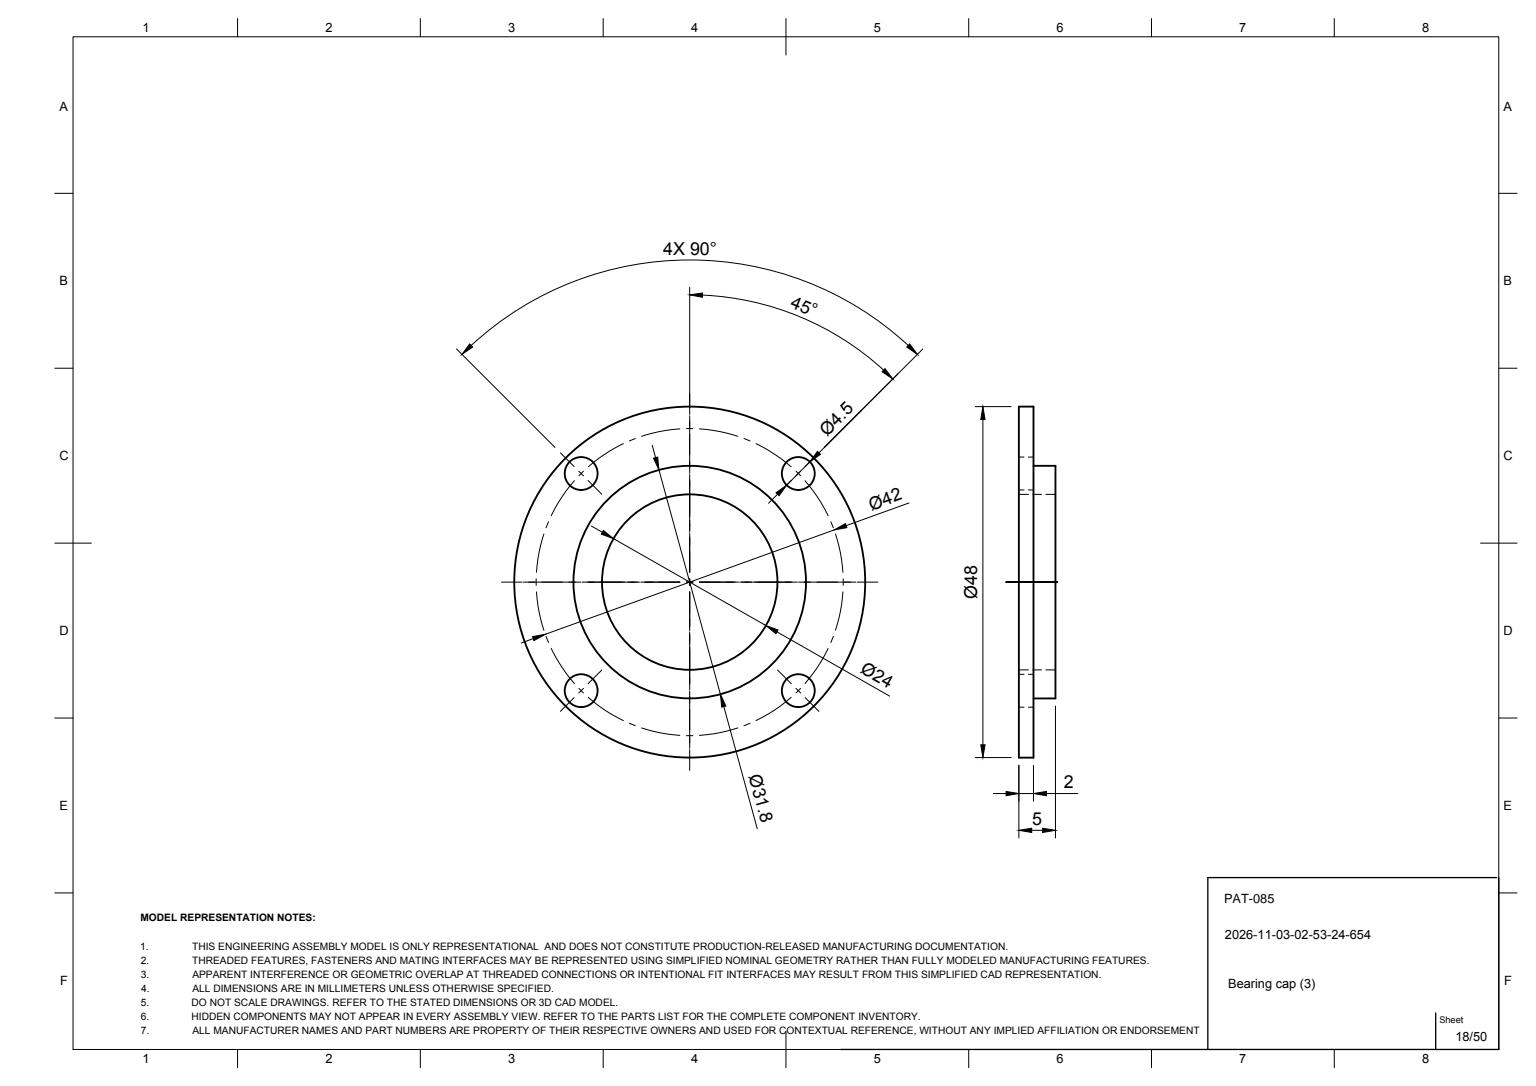
ISO-10303-21;
HEADER;
/* Generated by software containing ST-Developer
 * from STEP Tools, Inc. (www.steptools.com) 
 */

FILE_DESCRIPTION(
/* description */ ('Rack and pinion manual slide'),
/* implementation_level */ '2;1');

FILE_NAME(
/* name */ 'Bearing cap (3).step',
/* time_stamp */ '2026-10-28T03:22:49-07:00',
/* author */ (''),
/* organization */ (''),
/* preprocessor_version */ 'ST-DEVELOPER v20.2',
/* originating_system */ 'Autodesk Translation Framework v15.17.0.0',
/* authorisation */ '');

FILE_SCHEMA (('AUTOMOTIVE_DESIGN { 1 0 10303 214 3 1 1 }'));
ENDSEC;

DATA;
#10=MECHANICAL_DESIGN_GEOMETRIC_PRESENTATION_REPRESENTATION('',(#745),#34851);
#653=SHAPE_REPRESENTATION_RELATIONSHIP('SRR','None',#35088,#699);
#699=ADVANCED_BREP_SHAPE_REPRESENTATION('',(#798),#34813);
#745=STYLED_ITEM('',(#35411),#798);
#798=MANIFOLD_SOLID_BREP('Body1',#13765);
#946=FACE_BOUND('',#2537,.T.);
#947=FACE_BOUND('',#2541,.T.);
#948=FACE_BOUND('',#2542,.T.);
#949=FACE_BOUND('',#2543,.T.);
#950=FACE_BOUND('',#2544,.T.);
#951=FACE_BOUND('',#2545,.T.);
#952=FACE_BOUND('',#2547,.T.);
#953=FACE_BOUND('',#2548,.T.);
#954=FACE_BOUND('',#2549,.T.);
#955=FACE_BOUND('',#2550,.T.);
#956=FACE_BOUND('',#2551,.T.);
#1125=PLANE('',#14618);
#1126=PLANE('',#14625);
#1127=PLANE('',#14626);
#1679=FACE_OUTER_BOUND('',#2531,.T.);
#1680=FACE_OUTER_BOUND('',#2532,.T.);
#1681=FACE_OUTER_BOUND('',#2533,.T.);
#1682=FACE_OUTER_BOUND('',#2534,.T.);
#1683=FACE_OUTER_BOUND('',#2535,.T.);
#1684=FACE_OUTER_BOUND('',#2536,.T.);
#1685=FACE_OUTER_BOUND('',#2538,.T.);
#1686=FACE_OUTER_BOUND('',#2539,.T.);
#1687=FACE_OUTER_BOUND('',#2540,.T.);
#1688=FACE_OUTER_BOUND('',#2546,.T.);
#2531=EDGE_LOOP('',(#9900,#9901,#9902,#9903));
#2532=EDGE_LOOP('',(#9904,#9905,#9906,#9907));
#2533=EDGE_LOOP('',(#9908,#9909,#9910,#9911));
#2534=EDGE_LOOP('',(#9912,#9913,#9914,#9915));
#2535=EDGE_LOOP('',(#9916,#9917,#9918,#9919));
#2536=EDGE_LOOP('',(#9920));
#2537=EDGE_LOOP('',(#9921));
#2538=EDGE_LOOP('',(#9922,#9923,#9924,#9925));
#2539=EDGE_LOOP('',(#9926,#9927,#9928,#9929));
#2540=EDGE_LOOP('',(#9930));
#2541=EDGE_LOOP('',(#9931));
#2542=EDGE_LOOP('',(#9932));
#2543=EDGE_LOOP('',(#9933));
#2544=EDGE_LOOP('',(#9934));
#2545=EDGE_LOOP('',(#9935));
#2546=EDGE_LOOP('',(#9936));
#2547=EDGE_LOOP('',(#9937));
#2548=EDGE_LOOP('',(#9938));
#2549=EDGE_LOOP('',(#9939));
#2550=EDGE_LOOP('',(#9940));
#2551=EDGE_LOOP('',(#9941));
#3431=LINE('',#20176,#4722);
#3432=LINE('',#20182,#4723);
#3433=LINE('',#20188,#4724);
#3434=LINE('',#20194,#4725);
#3435=LINE('',#20200,#4726);
#3436=LINE('',#20208,#4727);
#3437=LINE('',#20213,#4728);
#4722=VECTOR('',#16383,0.225);
#4723=VECTOR('',#16390,0.225);
#4724=VECTOR('',#16397,0.225);
#4725=VECTOR('',#16404,0.225);
#4726=VECTOR('',#16411,1.59);
#4727=VECTOR('',#16422,1.2);
#4728=VECTOR('',#16427,2.4);
#5932=CIRCLE('',#14604,0.225);
#5933=CIRCLE('',#14605,0.225);
#5934=CIRCLE('',#14607,0.225);
#5935=CIRCLE('',#14608,0.225);
#5936=CIRCLE('',#14610,0.225);
#5937=CIRCLE('',#14611,0.225);
#5938=CIRCLE('',#14613,0.225);
#5939=CIRCLE('',#14614,0.225);
#5940=CIRCLE('',#14616,1.59);
#5941=CIRCLE('',#14617,1.59);
#5942=CIRCLE('',#14619,1.2);
#5943=CIRCLE('',#14621,1.2);
#5944=CIRCLE('',#14623,2.4);
#5945=CIRCLE('',#14624,2.4);
#6446=VERTEX_POINT('',#20173);
#6447=VERTEX_POINT('',#20175);
#6448=VERTEX_POINT('',#20179);
#6449=VERTEX_POINT('',#20181);
#6450=VERTEX_POINT('',#20185);
#6451=VERTEX_POINT('',#20187);
#6452=VERTEX_POINT('',#20191);
#6453=VERTEX_POINT('',#20193);
#6454=VERTEX_POINT('',#20197);
#6455=VERTEX_POINT('',#20199);
#6456=VERTEX_POINT('',#20203);
#6457=VERTEX_POINT('',#20206);
#6458=VERTEX_POINT('',#20210);
#6459=VERTEX_POINT('',#20212);
#7762=EDGE_CURVE('',#6446,#6446,#5932,.T.);
#7763=EDGE_CURVE('',#6446,#6447,#3431,.T.);
#7764=EDGE_CURVE('',#6447,#6447,#5933,.T.);
#7765=EDGE_CURVE('',#6448,#6448,#5934,.T.);
#7766=EDGE_CURVE('',#6448,#6449,#3432,.T.);
#7767=EDGE_CURVE('',#6449,#6449,#5935,.T.);
#7768=EDGE_CURVE('',#6450,#6450,#5936,.T.);
#7769=EDGE_CURVE('',#6450,#6451,#3433,.T.);
#7770=EDGE_CURVE('',#6451,#6451,#5937,.T.);
#7771=EDGE_CURVE('',#6452,#6452,#5938,.T.);
#7772=EDGE_CURVE('',#6452,#6453,#3434,.T.);
#7773=EDGE_CURVE('',#6453,#6453,#5939,.T.);
#7774=EDGE_CURVE('',#6454,#6454,#5940,.T.);
#7775=EDGE_CURVE('',#6454,#6455,#3435,.T.);
#7776=EDGE_CURVE('',#6455,#6455,#5941,.T.);
#7777=EDGE_CURVE('',#6456,#6456,#5942,.T.);
#7778=EDGE_CURVE('',#6457,#6457,#5943,.T.);
#7779=EDGE_CURVE('',#6457,#6456,#3436,.T.);
#7780=EDGE_CURVE('',#6458,#6458,#5944,.T.);
#7781=EDGE_CURVE('',#6458,#6459,#3437,.T.);
#7782=EDGE_CURVE('',#6459,#6459,#5945,.T.);
#9900=ORIENTED_EDGE('',*,*,#7762,.F.);
#9901=ORIENTED_EDGE('',*,*,#7763,.T.);
#9902=ORIENTED_EDGE('',*,*,#7764,.F.);
#9903=ORIENTED_EDGE('',*,*,#7763,.F.);
#9904=ORIENTED_EDGE('',*,*,#7765,.F.);
#9905=ORIENTED_EDGE('',*,*,#7766,.T.);
#9906=ORIENTED_EDGE('',*,*,#7767,.F.);
#9907=ORIENTED_EDGE('',*,*,#7766,.F.);
#9908=ORIENTED_EDGE('',*,*,#7768,.F.);
#9909=ORIENTED_EDGE('',*,*,#7769,.T.);
#9910=ORIENTED_EDGE('',*,*,#7770,.F.);
#9911=ORIENTED_EDGE('',*,*,#7769,.F.);
#9912=ORIENTED_EDGE('',*,*,#7771,.F.);
#9913=ORIENTED_EDGE('',*,*,#7772,.T.);
#9914=ORIENTED_EDGE('',*,*,#7773,.F.);
#9915=ORIENTED_EDGE('',*,*,#7772,.F.);
#9916=ORIENTED_EDGE('',*,*,#7774,.F.);
#9917=ORIENTED_EDGE('',*,*,#7775,.T.);
#9918=ORIENTED_EDGE('',*,*,#7776,.T.);
#9919=ORIENTED_EDGE('',*,*,#7775,.F.);
#9920=ORIENTED_EDGE('',*,*,#7776,.F.);
#9921=ORIENTED_EDGE('',*,*,#7777,.F.);
#9922=ORIENTED_EDGE('',*,*,#7778,.F.);
#9923=ORIENTED_EDGE('',*,*,#7779,.T.);
#9924=ORIENTED_EDGE('',*,*,#7777,.T.);
#9925=ORIENTED_EDGE('',*,*,#7779,.F.);
#9926=ORIENTED_EDGE('',*,*,#7780,.F.);
#9927=ORIENTED_EDGE('',*,*,#7781,.T.);
#9928=ORIENTED_EDGE('',*,*,#7782,.T.);
#9929=ORIENTED_EDGE('',*,*,#7781,.F.);
#9930=ORIENTED_EDGE('',*,*,#7780,.T.);
#9931=ORIENTED_EDGE('',*,*,#7778,.T.);
#9932=ORIENTED_EDGE('',*,*,#7773,.T.);
#9933=ORIENTED_EDGE('',*,*,#7770,.T.);
#9934=ORIENTED_EDGE('',*,*,#7767,.T.);
#9935=ORIENTED_EDGE('',*,*,#7764,.T.);
#9936=ORIENTED_EDGE('',*,*,#7782,.F.);
#9937=ORIENTED_EDGE('',*,*,#7774,.T.);
#9938=ORIENTED_EDGE('',*,*,#7771,.T.);
#9939=ORIENTED_EDGE('',*,*,#7768,.T.);
#9940=ORIENTED_EDGE('',*,*,#7765,.T.);
#9941=ORIENTED_EDGE('',*,*,#7762,.T.);
#12907=CYLINDRICAL_SURFACE('',#14603,0.225);
#12908=CYLINDRICAL_SURFACE('',#14606,0.225);
#12909=CYLINDRICAL_SURFACE('',#14609,0.225);
#12910=CYLINDRICAL_SURFACE('',#14612,0.225);
#12911=CYLINDRICAL_SURFACE('',#14615,1.59);
#12912=CYLINDRICAL_SURFACE('',#14620,1.2);
#12913=CYLINDRICAL_SURFACE('',#14622,2.4);
#13157=ADVANCED_FACE('',(#1679),#12907,.F.);
#13158=ADVANCED_FACE('',(#1680),#12908,.F.);
#13159=ADVANCED_FACE('',(#1681),#12909,.F.);
#13160=ADVANCED_FACE('',(#1682),#12910,.F.);
#13161=ADVANCED_FACE('',(#1683),#12911,.T.);
#13162=ADVANCED_FACE('',(#1684,#946),#1125,.F.);
#13163=ADVANCED_FACE('',(#1685),#12912,.F.);
#13164=ADVANCED_FACE('',(#1686),#12913,.T.);
#13165=ADVANCED_FACE('',(#1687,#947,#948,#949,#950,#951),#1126,.T.);
#13166=ADVANCED_FACE('',(#1688,#952,#953,#954,#955,#956),#1127,.F.);
#13765=CLOSED_SHELL('',(#13157,#13158,#13159,#13160,#13161,#13162,#13163,
#13164,#13165,#13166));
#14602=AXIS2_PLACEMENT_3D('',#20171,#16377,#16378);
#14603=AXIS2_PLACEMENT_3D('',#20172,#16379,#16380);
#14604=AXIS2_PLACEMENT_3D('',#20174,#16381,#16382);
#14605=AXIS2_PLACEMENT_3D('',#20177,#16384,#16385);
#14606=AXIS2_PLACEMENT_3D('',#20178,#16386,#16387);
#14607=AXIS2_PLACEMENT_3D('',#20180,#16388,#16389);
#14608=AXIS2_PLACEMENT_3D('',#20183,#16391,#16392);
#14609=AXIS2_PLACEMENT_3D('',#20184,#16393,#16394);
#14610=AXIS2_PLACEMENT_3D('',#20186,#16395,#16396);
#14611=AXIS2_PLACEMENT_3D('',#20189,#16398,#16399);
#14612=AXIS2_PLACEMENT_3D('',#20190,#16400,#16401);
#14613=AXIS2_PLACEMENT_3D('',#20192,#16402,#16403);
#14614=AXIS2_PLACEMENT_3D('',#20195,#16405,#16406);
#14615=AXIS2_PLACEMENT_3D('',#20196,#16407,#16408);
#14616=AXIS2_PLACEMENT_3D('',#20198,#16409,#16410);
#14617=AXIS2_PLACEMENT_3D('',#20201,#16412,#16413);
#14618=AXIS2_PLACEMENT_3D('',#20202,#16414,#16415);
#14619=AXIS2_PLACEMENT_3D('',#20204,#16416,#16417);
#14620=AXIS2_PLACEMENT_3D('',#20205,#16418,#16419);
#14621=AXIS2_PLACEMENT_3D('',#20207,#16420,#16421);
#14622=AXIS2_PLACEMENT_3D('',#20209,#16423,#16424);
#14623=AXIS2_PLACEMENT_3D('',#20211,#16425,#16426);
#14624=AXIS2_PLACEMENT_3D('',#20214,#16428,#16429);
#14625=AXIS2_PLACEMENT_3D('',#20215,#16430,#16431);
#14626=AXIS2_PLACEMENT_3D('',#20216,#16432,#16433);
#16377=DIRECTION('axis',(0.,0.,1.));
#16378=DIRECTION('refdir',(1.,0.,0.));
#16379=DIRECTION('center_axis',(0.,1.,0.));
#16380=DIRECTION('ref_axis',(1.,0.,0.));
#16381=DIRECTION('center_axis',(0.,1.,0.));
#16382=DIRECTION('ref_axis',(1.,0.,0.));
#16383=DIRECTION('',(0.,1.,0.));
#16384=DIRECTION('center_axis',(0.,-1.,0.));
#16385=DIRECTION('ref_axis',(1.,0.,0.));
#16386=DIRECTION('center_axis',(0.,1.,0.));
#16387=DIRECTION('ref_axis',(1.,0.,0.));
#16388=DIRECTION('center_axis',(0.,1.,0.));
#16389=DIRECTION('ref_axis',(1.,0.,0.));
#16390=DIRECTION('',(0.,1.,0.));
#16391=DIRECTION('center_axis',(0.,-1.,0.));
#16392=DIRECTION('ref_axis',(1.,0.,0.));
#16393=DIRECTION('center_axis',(0.,1.,0.));
#16394=DIRECTION('ref_axis',(1.,0.,0.));
#16395=DIRECTION('center_axis',(0.,1.,0.));
#16396=DIRECTION('ref_axis',(1.,0.,0.));
#16397=DIRECTION('',(0.,1.,0.));
#16398=DIRECTION('center_axis',(0.,-1.,0.));
#16399=DIRECTION('ref_axis',(1.,0.,0.));
#16400=DIRECTION('center_axis',(0.,1.,0.));
#16401=DIRECTION('ref_axis',(1.,0.,0.));
#16402=DIRECTION('center_axis',(0.,1.,0.));
#16403=DIRECTION('ref_axis',(1.,0.,0.));
#16404=DIRECTION('',(0.,1.,0.));
#16405=DIRECTION('center_axis',(0.,-1.,0.));
#16406=DIRECTION('ref_axis',(1.,0.,0.));
#16407=DIRECTION('center_axis',(0.,1.,0.));
#16408=DIRECTION('ref_axis',(1.,0.,0.));
#16409=DIRECTION('center_axis',(0.,1.,0.));
#16410=DIRECTION('ref_axis',(1.,0.,0.));
#16411=DIRECTION('',(0.,-1.,0.));
#16412=DIRECTION('center_axis',(0.,1.,0.));
#16413=DIRECTION('ref_axis',(1.,0.,0.));
#16414=DIRECTION('center_axis',(0.,1.,0.));
#16415=DIRECTION('ref_axis',(1.,0.,0.));
#16416=DIRECTION('center_axis',(0.,-1.,0.));
#16417=DIRECTION('ref_axis',(1.,0.,0.));
#16418=DIRECTION('center_axis',(0.,1.,0.));
#16419=DIRECTION('ref_axis',(1.,0.,0.));
#16420=DIRECTION('center_axis',(0.,-1.,0.));
#16421=DIRECTION('ref_axis',(1.,0.,0.));
#16422=DIRECTION('',(0.,-1.,0.));
#16423=DIRECTION('center_axis',(0.,1.,0.));
#16424=DIRECTION('ref_axis',(1.,0.,0.));
#16425=DIRECTION('center_axis',(0.,1.,0.));
#16426=DIRECTION('ref_axis',(1.,0.,0.));
#16427=DIRECTION('',(0.,-1.,0.));
#16428=DIRECTION('center_axis',(0.,1.,0.));
#16429=DIRECTION('ref_axis',(1.,0.,0.));
#16430=DIRECTION('center_axis',(0.,1.,0.));
#16431=DIRECTION('ref_axis',(1.,0.,0.));
#16432=DIRECTION('center_axis',(0.,1.,0.));
#16433=DIRECTION('ref_axis',(1.,0.,0.));
#20171=CARTESIAN_POINT('',(0.,0.,0.));
#20172=CARTESIAN_POINT('Origin',(9.51507575950825,4.9,8.76507575950825));
#20173=CARTESIAN_POINT('',(9.29007575950825,5.,8.76507575950825));
#20174=CARTESIAN_POINT('Origin',(9.51507575950825,5.,8.76507575950825));
#20175=CARTESIAN_POINT('',(9.29007575950825,5.2,8.76507575950825));
#20176=CARTESIAN_POINT('',(9.29007575950825,4.9,8.76507575950825));
#20177=CARTESIAN_POINT('Origin',(9.51507575950825,5.2,8.76507575950825));
#20178=CARTESIAN_POINT('Origin',(9.51507575950825,4.9,11.7349242404918));
#20179=CARTESIAN_POINT('',(9.29007575950825,5.,11.7349242404918));
#20180=CARTESIAN_POINT('Origin',(9.51507575950825,5.,11.7349242404918));
#20181=CARTESIAN_POINT('',(9.29007575950825,5.2,11.7349242404918));
#20182=CARTESIAN_POINT('',(9.29007575950825,4.9,11.7349242404918));
#20183=CARTESIAN_POINT('Origin',(9.51507575950825,5.2,11.7349242404918));
#20184=CARTESIAN_POINT('Origin',(12.4849242404918,4.9,11.7349242404918));
#20185=CARTESIAN_POINT('',(12.2599242404918,5.,11.7349242404918));
#20186=CARTESIAN_POINT('Origin',(12.4849242404918,5.,11.7349242404918));
#20187=CARTESIAN_POINT('',(12.2599242404918,5.2,11.7349242404918));
#20188=CARTESIAN_POINT('',(12.2599242404918,4.9,11.7349242404918));
#20189=CARTESIAN_POINT('Origin',(12.4849242404918,5.2,11.7349242404918));
#20190=CARTESIAN_POINT('Origin',(12.4849242404917,4.9,8.76507575950825));
#20191=CARTESIAN_POINT('',(12.2599242404917,5.,8.76507575950825));
#20192=CARTESIAN_POINT('Origin',(12.4849242404917,5.,8.76507575950825));
#20193=CARTESIAN_POINT('',(12.2599242404917,5.2,8.76507575950825));
#20194=CARTESIAN_POINT('',(12.2599242404917,4.9,8.76507575950825));
#20195=CARTESIAN_POINT('Origin',(12.4849242404917,5.2,8.76507575950825));
#20196=CARTESIAN_POINT('Origin',(11.,4.7,10.25));
#20197=CARTESIAN_POINT('',(9.41,5.,10.25));
#20198=CARTESIAN_POINT('Origin',(11.,5.,10.25));
#20199=CARTESIAN_POINT('',(9.41,4.7,10.25));
#20200=CARTESIAN_POINT('',(9.41,4.7,10.25));
#20201=CARTESIAN_POINT('Origin',(11.,4.7,10.25));
#20202=CARTESIAN_POINT('Origin',(11.,4.7,10.25));
#20203=CARTESIAN_POINT('',(9.8,4.7,10.25));
#20204=CARTESIAN_POINT('Origin',(11.,4.7,10.25));
#20205=CARTESIAN_POINT('Origin',(11.,5.,10.25));
#20206=CARTESIAN_POINT('',(9.8,5.2,10.25));
#20207=CARTESIAN_POINT('Origin',(11.,5.2,10.25));
#20208=CARTESIAN_POINT('',(9.8,5.,10.25));
#20209=CARTESIAN_POINT('Origin',(11.,5.,10.25));
#20210=CARTESIAN_POINT('',(8.6,5.2,10.25));
#20211=CARTESIAN_POINT('Origin',(11.,5.2,10.25));
#20212=CARTESIAN_POINT('',(8.6,5.,10.25));
#20213=CARTESIAN_POINT('',(8.6,5.,10.25));
#20214=CARTESIAN_POINT('Origin',(11.,5.,10.25));
#20215=CARTESIAN_POINT('Origin',(11.,5.2,10.25));
#20216=CARTESIAN_POINT('Origin',(11.,5.,10.25));
#34759=UNCERTAINTY_MEASURE_WITH_UNIT(LENGTH_MEASURE(0.001),#34852,
'DISTANCE_ACCURACY_VALUE',
'Maximum model space distance between geometric entities at asserted c
onnectivities');
#34797=UNCERTAINTY_MEASURE_WITH_UNIT(LENGTH_MEASURE(0.001),#34852,
'DISTANCE_ACCURACY_VALUE',
'Maximum model space distance between geometric entities at asserted c
onnectivities');
#34813=(
GEOMETRIC_REPRESENTATION_CONTEXT(3)
GLOBAL_UNCERTAINTY_ASSIGNED_CONTEXT((#34759))
GLOBAL_UNIT_ASSIGNED_CONTEXT((#34852,#34854,#34855))
REPRESENTATION_CONTEXT('','3D')
);
#34851=(
GEOMETRIC_REPRESENTATION_CONTEXT(3)
GLOBAL_UNCERTAINTY_ASSIGNED_CONTEXT((#34797))
GLOBAL_UNIT_ASSIGNED_CONTEXT((#34852,#34854,#34855))
REPRESENTATION_CONTEXT('','3D')
);
#34852=(
LENGTH_UNIT()
NAMED_UNIT(*)
SI_UNIT(.CENTI.,.METRE.)
);
#34854=(
NAMED_UNIT(*)
PLANE_ANGLE_UNIT()
SI_UNIT($,.RADIAN.)
);
#34855=(
NAMED_UNIT(*)
SI_UNIT($,.STERADIAN.)
SOLID_ANGLE_UNIT()
);
#34871=SHAPE_DEFINITION_REPRESENTATION(#34924,#35088);
#34924=PRODUCT_DEFINITION_SHAPE('',$,#35142);
#35088=SHAPE_REPRESENTATION('',(#14602),#34813);
#35126=PRODUCT_DEFINITION_CONTEXT('part definition',#35287,'design');
#35142=PRODUCT_DEFINITION('Bearing cap (3)','Bearing cap (3)',#35195,#35126);
#35195=PRODUCT_DEFINITION_FORMATION('',$,#35304);
#35287=APPLICATION_CONTEXT(
'Core Data for Automotive Mechanical Design Process');
#35288=PRODUCT_CONTEXT('part definition',#35287,'mechanical');
#35304=PRODUCT('Bearing cap (3)','Bearing cap (3)','Bearing cap (3)',(#35288));
#35405=COLOUR_RGB('Grey',0.48,0.52,0.57);
#35406=FILL_AREA_STYLE_COLOUR('',#35405);
#35407=FILL_AREA_STYLE('',(#35406));
#35408=SURFACE_STYLE_FILL_AREA(#35407);
#35409=SURFACE_SIDE_STYLE('',(#35408));
#35410=SURFACE_STYLE_USAGE(.BOTH.,#35409);
#35411=PRESENTATION_STYLE_ASSIGNMENT((#35410));
ENDSEC;
END-ISO-10303-21;
